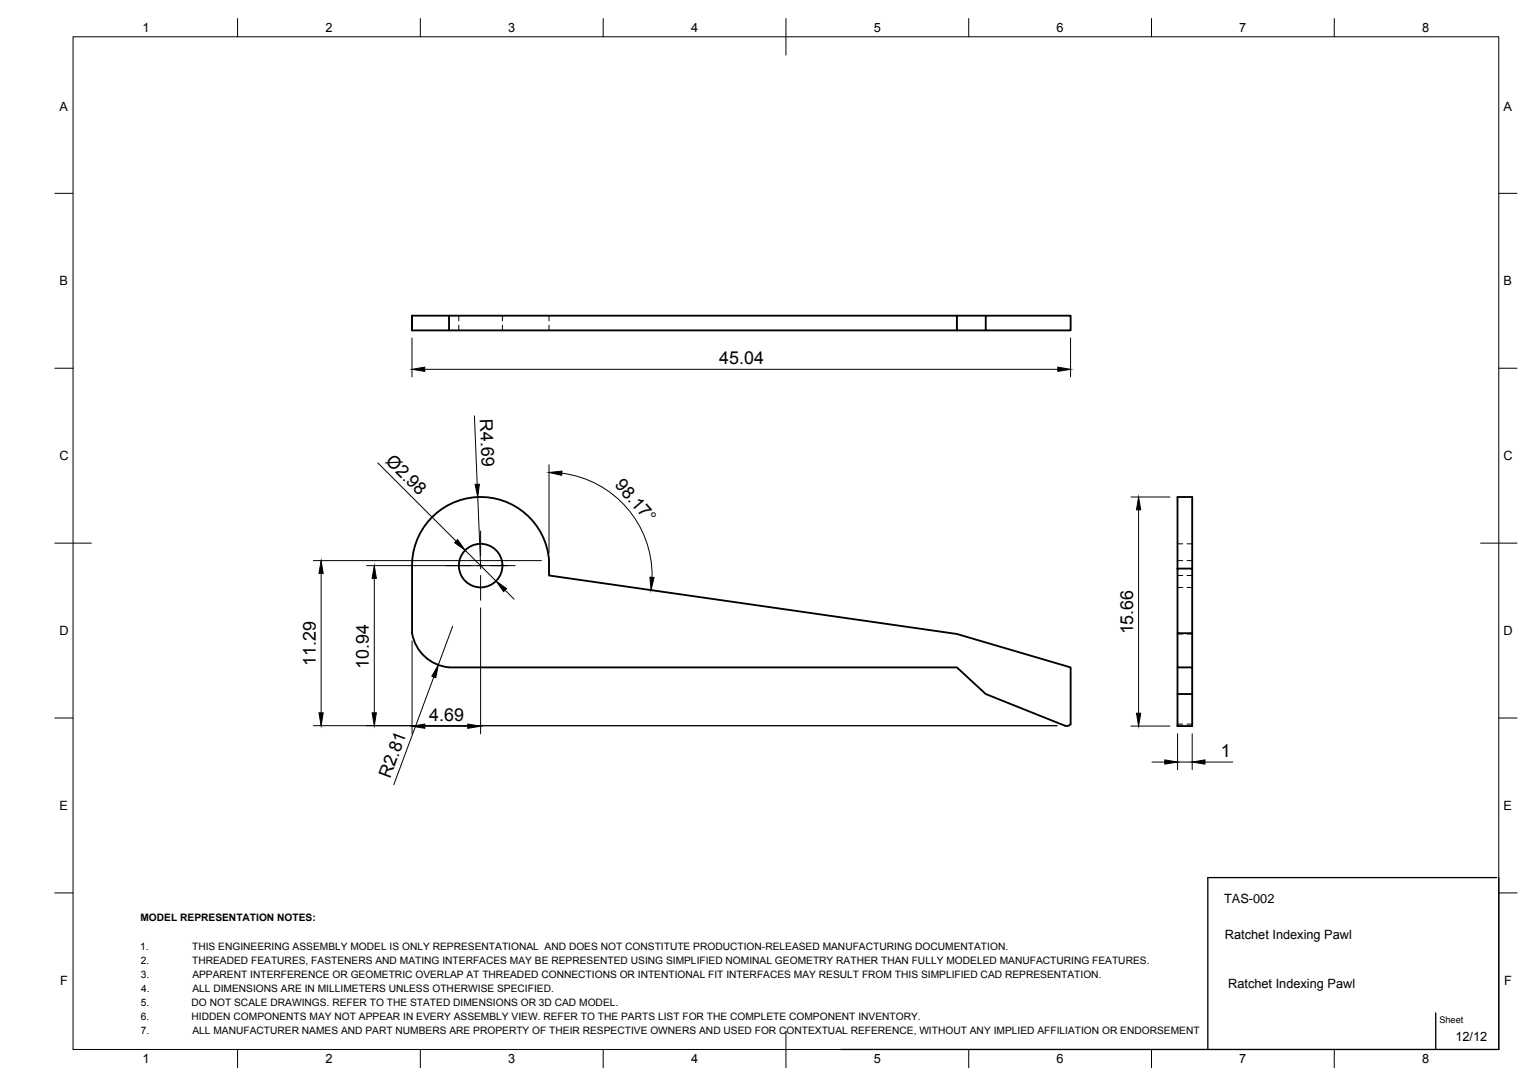
ISO-10303-21;
HEADER;
/* Generated by software containing ST-Developer
 * from STEP Tools, Inc. (www.steptools.com) 
 */

FILE_DESCRIPTION(
/* description */ ('STEP AP214'),
/* implementation_level */ '2;1');

FILE_NAME(
/* name */ 'Ratchet Indexing Pawl.step',
/* time_stamp */ '2026-11-04T19:38:14-08:00',
/* author */ (''),
/* organization */ (''),
/* preprocessor_version */ 'ST-DEVELOPER v20.2',
/* originating_system */ 'Autodesk Translation Framework v15.17.0.0',
/* authorisation */ '');

FILE_SCHEMA (('AUTOMOTIVE_DESIGN { 1 0 10303 214 3 1 1 }'));
ENDSEC;

DATA;
#10=MECHANICAL_DESIGN_GEOMETRIC_PRESENTATION_REPRESENTATION('',(#479),#36668);
#459=SHAPE_REPRESENTATION_RELATIONSHIP('SRR','None',#36715,#469);
#469=ADVANCED_BREP_SHAPE_REPRESENTATION('',(#488),#36667);
#479=STYLED_ITEM('',(#36766),#488);
#488=MANIFOLD_SOLID_BREP('Body1',#17803);
#772=CYLINDRICAL_SURFACE('',#19406,1.49172584788676);
#773=CYLINDRICAL_SURFACE('',#19410,4.6918515041613);
#774=CYLINDRICAL_SURFACE('',#19417,0.338583852498097);
#775=CYLINDRICAL_SURFACE('',#19423,2.81299719163292);
#971=FACE_BOUND('',#3583,.T.);
#972=FACE_BOUND('',#3585,.T.);
#1519=CIRCLE('',#19407,1.49172584788676);
#1520=CIRCLE('',#19408,1.49172584788676);
#1521=CIRCLE('',#19411,4.6918515041613);
#1522=CIRCLE('',#19412,4.6918515041613);
#1523=CIRCLE('',#19418,0.338583852498097);
#1524=CIRCLE('',#19419,0.338583852498097);
#1525=CIRCLE('',#19424,2.81299719163292);
#1526=CIRCLE('',#19425,2.81299719163292);
#2444=FACE_OUTER_BOUND('',#3570,.T.);
#2445=FACE_OUTER_BOUND('',#3571,.T.);
#2446=FACE_OUTER_BOUND('',#3572,.T.);
#2447=FACE_OUTER_BOUND('',#3573,.T.);
#2448=FACE_OUTER_BOUND('',#3574,.T.);
#2449=FACE_OUTER_BOUND('',#3575,.T.);
#2450=FACE_OUTER_BOUND('',#3576,.T.);
#2451=FACE_OUTER_BOUND('',#3577,.T.);
#2452=FACE_OUTER_BOUND('',#3578,.T.);
#2453=FACE_OUTER_BOUND('',#3579,.T.);
#2454=FACE_OUTER_BOUND('',#3580,.T.);
#2455=FACE_OUTER_BOUND('',#3581,.T.);
#2456=FACE_OUTER_BOUND('',#3582,.T.);
#2457=FACE_OUTER_BOUND('',#3584,.T.);
#3570=EDGE_LOOP('',(#16252,#16253,#16254,#16255));
#3571=EDGE_LOOP('',(#16256,#16257,#16258,#16259));
#3572=EDGE_LOOP('',(#16260,#16261,#16262,#16263));
#3573=EDGE_LOOP('',(#16264,#16265,#16266,#16267));
#3574=EDGE_LOOP('',(#16268,#16269,#16270,#16271));
#3575=EDGE_LOOP('',(#16272,#16273,#16274,#16275));
#3576=EDGE_LOOP('',(#16276,#16277,#16278,#16279));
#3577=EDGE_LOOP('',(#16280,#16281,#16282,#16283));
#3578=EDGE_LOOP('',(#16284,#16285,#16286,#16287));
#3579=EDGE_LOOP('',(#16288,#16289,#16290,#16291));
#3580=EDGE_LOOP('',(#16292,#16293,#16294,#16295));
#3581=EDGE_LOOP('',(#16296,#16297,#16298,#16299));
#3582=EDGE_LOOP('',(#16300,#16301,#16302,#16303,#16304,#16305,#16306,#16307,
#16308,#16309,#16310));
#3583=EDGE_LOOP('',(#16311));
#3584=EDGE_LOOP('',(#16312,#16313,#16314,#16315,#16316,#16317,#16318,#16319,
#16320,#16321,#16322));
#3585=EDGE_LOOP('',(#16323));
#5268=LINE('',#36565,#6978);
#5269=LINE('',#36570,#6979);
#5270=LINE('',#36572,#6980);
#5271=LINE('',#36574,#6981);
#5272=LINE('',#36575,#6982);
#5273=LINE('',#36580,#6983);
#5274=LINE('',#36584,#6984);
#5275=LINE('',#36586,#6985);
#5276=LINE('',#36587,#6986);
#5277=LINE('',#36590,#6987);
#5278=LINE('',#36592,#6988);
#5279=LINE('',#36593,#6989);
#5280=LINE('',#36596,#6990);
#5281=LINE('',#36598,#6991);
#5282=LINE('',#36599,#6992);
#5283=LINE('',#36602,#6993);
#5284=LINE('',#36604,#6994);
#5285=LINE('',#36605,#6995);
#5286=LINE('',#36611,#6996);
#5287=LINE('',#36614,#6997);
#5288=LINE('',#36616,#6998);
#5289=LINE('',#36617,#6999);
#5290=LINE('',#36620,#7000);
#5291=LINE('',#36622,#7001);
#5292=LINE('',#36623,#7002);
#5293=LINE('',#36626,#7003);
#5294=LINE('',#36628,#7004);
#5295=LINE('',#36629,#7005);
#6978=VECTOR('',#24106,1.49172584788676);
#6979=VECTOR('',#24111,1000.);
#6980=VECTOR('',#24112,1000.);
#6981=VECTOR('',#24113,1000.);
#6982=VECTOR('',#24114,1000.);
#6983=VECTOR('',#24119,1000.);
#6984=VECTOR('',#24124,1000.);
#6985=VECTOR('',#24125,1000.);
#6986=VECTOR('',#24126,1000.);
#6987=VECTOR('',#24129,1000.);
#6988=VECTOR('',#24130,1000.);
#6989=VECTOR('',#24131,1000.);
#6990=VECTOR('',#24134,1000.);
#6991=VECTOR('',#24135,1000.);
#6992=VECTOR('',#24136,1000.);
#6993=VECTOR('',#24139,1000.);
#6994=VECTOR('',#24140,1000.);
#6995=VECTOR('',#24141,1000.);
#6996=VECTOR('',#24148,1000.);
#6997=VECTOR('',#24151,1000.);
#6998=VECTOR('',#24152,1000.);
#6999=VECTOR('',#24153,1000.);
#7000=VECTOR('',#24156,1000.);
#7001=VECTOR('',#24157,1000.);
#7002=VECTOR('',#24158,1000.);
#7003=VECTOR('',#24161,1000.);
#7004=VECTOR('',#24162,1000.);
#7005=VECTOR('',#24163,1000.);
#8635=VERTEX_POINT('',#36562);
#8636=VERTEX_POINT('',#36564);
#8637=VERTEX_POINT('',#36568);
#8638=VERTEX_POINT('',#36569);
#8639=VERTEX_POINT('',#36571);
#8640=VERTEX_POINT('',#36573);
#8641=VERTEX_POINT('',#36577);
#8642=VERTEX_POINT('',#36579);
#8643=VERTEX_POINT('',#36583);
#8644=VERTEX_POINT('',#36585);
#8645=VERTEX_POINT('',#36589);
#8646=VERTEX_POINT('',#36591);
#8647=VERTEX_POINT('',#36595);
#8648=VERTEX_POINT('',#36597);
#8649=VERTEX_POINT('',#36601);
#8650=VERTEX_POINT('',#36603);
#8651=VERTEX_POINT('',#36607);
#8652=VERTEX_POINT('',#36609);
#8653=VERTEX_POINT('',#36613);
#8654=VERTEX_POINT('',#36615);
#8655=VERTEX_POINT('',#36619);
#8656=VERTEX_POINT('',#36621);
#8657=VERTEX_POINT('',#36625);
#8658=VERTEX_POINT('',#36627);
#11178=EDGE_CURVE('',#8635,#8635,#1519,.T.);
#11179=EDGE_CURVE('',#8635,#8636,#5268,.T.);
#11180=EDGE_CURVE('',#8636,#8636,#1520,.T.);
#11181=EDGE_CURVE('',#8637,#8638,#5269,.T.);
#11182=EDGE_CURVE('',#8639,#8638,#5270,.T.);
#11183=EDGE_CURVE('',#8640,#8639,#5271,.T.);
#11184=EDGE_CURVE('',#8640,#8637,#5272,.T.);
#11185=EDGE_CURVE('',#8641,#8640,#1521,.T.);
#11186=EDGE_CURVE('',#8641,#8642,#5273,.T.);
#11187=EDGE_CURVE('',#8642,#8637,#1522,.T.);
#11188=EDGE_CURVE('',#8643,#8642,#5274,.T.);
#11189=EDGE_CURVE('',#8644,#8641,#5275,.T.);
#11190=EDGE_CURVE('',#8644,#8643,#5276,.T.);
#11191=EDGE_CURVE('',#8645,#8643,#5277,.T.);
#11192=EDGE_CURVE('',#8646,#8644,#5278,.T.);
#11193=EDGE_CURVE('',#8646,#8645,#5279,.T.);
#11194=EDGE_CURVE('',#8647,#8645,#5280,.T.);
#11195=EDGE_CURVE('',#8648,#8646,#5281,.T.);
#11196=EDGE_CURVE('',#8648,#8647,#5282,.T.);
#11197=EDGE_CURVE('',#8649,#8647,#5283,.T.);
#11198=EDGE_CURVE('',#8650,#8648,#5284,.T.);
#11199=EDGE_CURVE('',#8650,#8649,#5285,.T.);
#11200=EDGE_CURVE('',#8651,#8649,#1523,.T.);
#11201=EDGE_CURVE('',#8652,#8650,#1524,.T.);
#11202=EDGE_CURVE('',#8652,#8651,#5286,.T.);
#11203=EDGE_CURVE('',#8653,#8651,#5287,.T.);
#11204=EDGE_CURVE('',#8654,#8652,#5288,.T.);
#11205=EDGE_CURVE('',#8654,#8653,#5289,.T.);
#11206=EDGE_CURVE('',#8655,#8653,#5290,.T.);
#11207=EDGE_CURVE('',#8656,#8654,#5291,.T.);
#11208=EDGE_CURVE('',#8656,#8655,#5292,.T.);
#11209=EDGE_CURVE('',#8657,#8655,#5293,.T.);
#11210=EDGE_CURVE('',#8658,#8656,#5294,.T.);
#11211=EDGE_CURVE('',#8658,#8657,#5295,.T.);
#11212=EDGE_CURVE('',#8638,#8657,#1525,.T.);
#11213=EDGE_CURVE('',#8639,#8658,#1526,.T.);
#16252=ORIENTED_EDGE('',*,*,#11178,.T.);
#16253=ORIENTED_EDGE('',*,*,#11179,.T.);
#16254=ORIENTED_EDGE('',*,*,#11180,.T.);
#16255=ORIENTED_EDGE('',*,*,#11179,.F.);
#16256=ORIENTED_EDGE('',*,*,#11181,.T.);
#16257=ORIENTED_EDGE('',*,*,#11182,.F.);
#16258=ORIENTED_EDGE('',*,*,#11183,.F.);
#16259=ORIENTED_EDGE('',*,*,#11184,.T.);
#16260=ORIENTED_EDGE('',*,*,#11185,.F.);
#16261=ORIENTED_EDGE('',*,*,#11186,.T.);
#16262=ORIENTED_EDGE('',*,*,#11187,.T.);
#16263=ORIENTED_EDGE('',*,*,#11184,.F.);
#16264=ORIENTED_EDGE('',*,*,#11188,.T.);
#16265=ORIENTED_EDGE('',*,*,#11186,.F.);
#16266=ORIENTED_EDGE('',*,*,#11189,.F.);
#16267=ORIENTED_EDGE('',*,*,#11190,.T.);
#16268=ORIENTED_EDGE('',*,*,#11191,.T.);
#16269=ORIENTED_EDGE('',*,*,#11190,.F.);
#16270=ORIENTED_EDGE('',*,*,#11192,.F.);
#16271=ORIENTED_EDGE('',*,*,#11193,.T.);
#16272=ORIENTED_EDGE('',*,*,#11194,.T.);
#16273=ORIENTED_EDGE('',*,*,#11193,.F.);
#16274=ORIENTED_EDGE('',*,*,#11195,.F.);
#16275=ORIENTED_EDGE('',*,*,#11196,.T.);
#16276=ORIENTED_EDGE('',*,*,#11197,.T.);
#16277=ORIENTED_EDGE('',*,*,#11196,.F.);
#16278=ORIENTED_EDGE('',*,*,#11198,.F.);
#16279=ORIENTED_EDGE('',*,*,#11199,.T.);
#16280=ORIENTED_EDGE('',*,*,#11200,.T.);
#16281=ORIENTED_EDGE('',*,*,#11199,.F.);
#16282=ORIENTED_EDGE('',*,*,#11201,.F.);
#16283=ORIENTED_EDGE('',*,*,#11202,.T.);
#16284=ORIENTED_EDGE('',*,*,#11203,.T.);
#16285=ORIENTED_EDGE('',*,*,#11202,.F.);
#16286=ORIENTED_EDGE('',*,*,#11204,.F.);
#16287=ORIENTED_EDGE('',*,*,#11205,.T.);
#16288=ORIENTED_EDGE('',*,*,#11206,.T.);
#16289=ORIENTED_EDGE('',*,*,#11205,.F.);
#16290=ORIENTED_EDGE('',*,*,#11207,.F.);
#16291=ORIENTED_EDGE('',*,*,#11208,.T.);
#16292=ORIENTED_EDGE('',*,*,#11209,.T.);
#16293=ORIENTED_EDGE('',*,*,#11208,.F.);
#16294=ORIENTED_EDGE('',*,*,#11210,.F.);
#16295=ORIENTED_EDGE('',*,*,#11211,.T.);
#16296=ORIENTED_EDGE('',*,*,#11212,.T.);
#16297=ORIENTED_EDGE('',*,*,#11211,.F.);
#16298=ORIENTED_EDGE('',*,*,#11213,.F.);
#16299=ORIENTED_EDGE('',*,*,#11182,.T.);
#16300=ORIENTED_EDGE('',*,*,#11212,.F.);
#16301=ORIENTED_EDGE('',*,*,#11181,.F.);
#16302=ORIENTED_EDGE('',*,*,#11187,.F.);
#16303=ORIENTED_EDGE('',*,*,#11188,.F.);
#16304=ORIENTED_EDGE('',*,*,#11191,.F.);
#16305=ORIENTED_EDGE('',*,*,#11194,.F.);
#16306=ORIENTED_EDGE('',*,*,#11197,.F.);
#16307=ORIENTED_EDGE('',*,*,#11200,.F.);
#16308=ORIENTED_EDGE('',*,*,#11203,.F.);
#16309=ORIENTED_EDGE('',*,*,#11206,.F.);
#16310=ORIENTED_EDGE('',*,*,#11209,.F.);
#16311=ORIENTED_EDGE('',*,*,#11178,.F.);
#16312=ORIENTED_EDGE('',*,*,#11213,.T.);
#16313=ORIENTED_EDGE('',*,*,#11210,.T.);
#16314=ORIENTED_EDGE('',*,*,#11207,.T.);
#16315=ORIENTED_EDGE('',*,*,#11204,.T.);
#16316=ORIENTED_EDGE('',*,*,#11201,.T.);
#16317=ORIENTED_EDGE('',*,*,#11198,.T.);
#16318=ORIENTED_EDGE('',*,*,#11195,.T.);
#16319=ORIENTED_EDGE('',*,*,#11192,.T.);
#16320=ORIENTED_EDGE('',*,*,#11189,.T.);
#16321=ORIENTED_EDGE('',*,*,#11185,.T.);
#16322=ORIENTED_EDGE('',*,*,#11183,.T.);
#16323=ORIENTED_EDGE('',*,*,#11180,.F.);
#16852=PLANE('',#19409);
#16853=PLANE('',#19413);
#16854=PLANE('',#19414);
#16855=PLANE('',#19415);
#16856=PLANE('',#19416);
#16857=PLANE('',#19420);
#16858=PLANE('',#19421);
#16859=PLANE('',#19422);
#16860=PLANE('',#19426);
#16861=PLANE('',#19427);
#17779=ADVANCED_FACE('',(#2444),#772,.F.);
#17780=ADVANCED_FACE('',(#2445),#16852,.F.);
#17781=ADVANCED_FACE('',(#2446),#773,.T.);
#17782=ADVANCED_FACE('',(#2447),#16853,.F.);
#17783=ADVANCED_FACE('',(#2448),#16854,.F.);
#17784=ADVANCED_FACE('',(#2449),#16855,.F.);
#17785=ADVANCED_FACE('',(#2450),#16856,.F.);
#17786=ADVANCED_FACE('',(#2451),#774,.T.);
#17787=ADVANCED_FACE('',(#2452),#16857,.F.);
#17788=ADVANCED_FACE('',(#2453),#16858,.F.);
#17789=ADVANCED_FACE('',(#2454),#16859,.F.);
#17790=ADVANCED_FACE('',(#2455),#775,.T.);
#17791=ADVANCED_FACE('',(#2456,#971),#16860,.T.);
#17792=ADVANCED_FACE('',(#2457,#972),#16861,.F.);
#17803=CLOSED_SHELL('',(#17779,#17780,#17781,#17782,#17783,#17784,#17785,
#17786,#17787,#17788,#17789,#17790,#17791,#17792));
#19405=AXIS2_PLACEMENT_3D('',#36560,#24100,#24101);
#19406=AXIS2_PLACEMENT_3D('',#36561,#24102,#24103);
#19407=AXIS2_PLACEMENT_3D('',#36563,#24104,#24105);
#19408=AXIS2_PLACEMENT_3D('',#36566,#24107,#24108);
#19409=AXIS2_PLACEMENT_3D('',#36567,#24109,#24110);
#19410=AXIS2_PLACEMENT_3D('',#36576,#24115,#24116);
#19411=AXIS2_PLACEMENT_3D('',#36578,#24117,#24118);
#19412=AXIS2_PLACEMENT_3D('',#36581,#24120,#24121);
#19413=AXIS2_PLACEMENT_3D('',#36582,#24122,#24123);
#19414=AXIS2_PLACEMENT_3D('',#36588,#24127,#24128);
#19415=AXIS2_PLACEMENT_3D('',#36594,#24132,#24133);
#19416=AXIS2_PLACEMENT_3D('',#36600,#24137,#24138);
#19417=AXIS2_PLACEMENT_3D('',#36606,#24142,#24143);
#19418=AXIS2_PLACEMENT_3D('',#36608,#24144,#24145);
#19419=AXIS2_PLACEMENT_3D('',#36610,#24146,#24147);
#19420=AXIS2_PLACEMENT_3D('',#36612,#24149,#24150);
#19421=AXIS2_PLACEMENT_3D('',#36618,#24154,#24155);
#19422=AXIS2_PLACEMENT_3D('',#36624,#24159,#24160);
#19423=AXIS2_PLACEMENT_3D('',#36630,#24164,#24165);
#19424=AXIS2_PLACEMENT_3D('',#36631,#24166,#24167);
#19425=AXIS2_PLACEMENT_3D('',#36632,#24168,#24169);
#19426=AXIS2_PLACEMENT_3D('',#36633,#24170,#24171);
#19427=AXIS2_PLACEMENT_3D('',#36634,#24172,#24173);
#24100=DIRECTION('axis',(0.,0.,1.));
#24101=DIRECTION('refdir',(1.,0.,0.));
#24102=DIRECTION('center_axis',(0.,0.,-1.));
#24103=DIRECTION('ref_axis',(-1.,0.,0.));
#24104=DIRECTION('center_axis',(0.,0.,1.));
#24105=DIRECTION('ref_axis',(1.,0.,0.));
#24106=DIRECTION('',(0.,0.,-1.));
#24107=DIRECTION('center_axis',(0.,0.,-1.));
#24108=DIRECTION('ref_axis',(-1.,0.,0.));
#24109=DIRECTION('center_axis',(-0.999428214444506,-0.033811893946752,0.));
#24110=DIRECTION('ref_axis',(-0.033811893946752,0.999428214444506,0.));
#24111=DIRECTION('',(0.033811893946752,-0.999428214444506,0.));
#24112=DIRECTION('',(0.,0.,1.));
#24113=DIRECTION('',(0.033811893946752,-0.999428214444506,0.));
#24114=DIRECTION('',(0.,0.,1.));
#24115=DIRECTION('center_axis',(0.,0.,1.));
#24116=DIRECTION('ref_axis',(0.999428214444506,0.0338118939467526,0.));
#24117=DIRECTION('center_axis',(0.,0.,-1.));
#24118=DIRECTION('ref_axis',(0.999428214444506,0.0338118939467526,0.));
#24119=DIRECTION('',(0.,0.,1.));
#24120=DIRECTION('center_axis',(0.,0.,-1.));
#24121=DIRECTION('ref_axis',(0.999428214444506,0.0338118939467526,0.));
#24122=DIRECTION('center_axis',(0.999428214444506,0.0338118939467537,0.));
#24123=DIRECTION('ref_axis',(0.,0.,-1.));
#24124=DIRECTION('',(-0.0338118939467537,0.999428214444506,0.));
#24125=DIRECTION('',(-0.0338118939467537,0.999428214444506,0.));
#24126=DIRECTION('',(0.,0.,1.));
#24127=DIRECTION('center_axis',(0.175442327597817,-0.984489710300245,0.));
#24128=DIRECTION('ref_axis',(0.984489710300245,0.175442327597816,0.));
#24129=DIRECTION('',(0.984489710300245,0.175442327597816,0.));
#24130=DIRECTION('',(0.984489710300248,0.1754423275978,0.));
#24131=DIRECTION('',(0.,0.,1.));
#24132=DIRECTION('center_axis',(0.314024880544539,-0.949414753624036,0.));
#24133=DIRECTION('ref_axis',(0.949414753624036,0.314024880544539,0.));
#24134=DIRECTION('',(0.949414753624036,0.314024880544539,0.));
#24135=DIRECTION('',(0.949414753624036,0.314024880544539,0.));
#24136=DIRECTION('',(0.,0.,1.));
#24137=DIRECTION('center_axis',(0.999428214444506,0.033811893946752,0.));
#24138=DIRECTION('ref_axis',(0.,0.,-1.));
#24139=DIRECTION('',(-0.033811893946752,0.999428214444506,0.));
#24140=DIRECTION('',(-0.033811893946752,0.999428214444506,0.));
#24141=DIRECTION('',(0.,0.,1.));
#24142=DIRECTION('center_axis',(0.,0.,1.));
#24143=DIRECTION('ref_axis',(0.999428214444506,0.0338118939467424,0.));
#24144=DIRECTION('center_axis',(0.,0.,-1.));
#24145=DIRECTION('ref_axis',(0.999428214444506,0.0338118939467424,0.));
#24146=DIRECTION('center_axis',(0.,0.,-1.));
#24147=DIRECTION('ref_axis',(0.999428214444506,0.0338118939467424,0.));
#24148=DIRECTION('',(0.,0.,1.));
#24149=DIRECTION('center_axis',(-0.40290063302029,0.915243727054084,0.));
#24150=DIRECTION('ref_axis',(0.,0.,1.));
#24151=DIRECTION('',(-0.915243727054084,-0.402900633020289,0.));
#24152=DIRECTION('',(-0.915243727054084,-0.402900633020289,0.));
#24153=DIRECTION('',(0.,0.,1.));
#24154=DIRECTION('center_axis',(-0.702321846847344,0.711859553171084,0.));
#24155=DIRECTION('ref_axis',(0.,0.,1.));
#24156=DIRECTION('',(-0.711859553171084,-0.702321846847344,0.));
#24157=DIRECTION('',(-0.711859553171084,-0.702321846847344,0.));
#24158=DIRECTION('',(0.,0.,1.));
#24159=DIRECTION('center_axis',(-0.033811893946752,0.999428214444506,0.));
#24160=DIRECTION('ref_axis',(-0.999428214444506,-0.033811893946752,0.));
#24161=DIRECTION('',(-0.999428214444506,-0.033811893946752,0.));
#24162=DIRECTION('',(-0.999428214444506,-0.033811893946752,0.));
#24163=DIRECTION('',(0.,0.,1.));
#24164=DIRECTION('center_axis',(0.,0.,1.));
#24165=DIRECTION('ref_axis',(0.999428214444506,0.0338118939467518,0.));
#24166=DIRECTION('center_axis',(0.,0.,-1.));
#24167=DIRECTION('ref_axis',(0.999428214444506,0.0338118939467518,0.));
#24168=DIRECTION('center_axis',(0.,0.,-1.));
#24169=DIRECTION('ref_axis',(0.999428214444506,0.0338118939467518,0.));
#24170=DIRECTION('center_axis',(0.,0.,1.));
#24171=DIRECTION('ref_axis',(0.033811893946752,-0.999428214444506,0.));
#24172=DIRECTION('center_axis',(0.,0.,1.));
#24173=DIRECTION('ref_axis',(0.033811893946752,-0.999428214444506,0.));
#36560=CARTESIAN_POINT('',(0.,0.,0.));
#36561=CARTESIAN_POINT('Origin',(19.9513700273636,43.5818784659284,216.094898865397));
#36562=CARTESIAN_POINT('',(21.4430958752503,43.5818784659284,209.094898865397));
#36563=CARTESIAN_POINT('Origin',(19.9513700273636,43.5818784659284,209.094898865397));
#36564=CARTESIAN_POINT('',(21.4430958752503,43.5818784659284,208.094898865397));
#36565=CARTESIAN_POINT('',(21.4430958752503,43.5818784659284,216.094898865397));
#36566=CARTESIAN_POINT('Origin',(19.9513700273636,43.5818784659284,208.094898865397));
#36567=CARTESIAN_POINT('Origin',(24.6430224985391,43.5386624163653,208.094898865397));
#36568=CARTESIAN_POINT('',(24.6430224985391,43.5386624163653,209.094898865397));
#36569=CARTESIAN_POINT('',(24.7923296637165,39.1253694570289,209.094898865397));
#36570=CARTESIAN_POINT('',(24.6430224985391,43.5386624163653,209.094898865397));
#36571=CARTESIAN_POINT('',(24.7923296637165,39.1253694570289,208.094898865397));
#36572=CARTESIAN_POINT('',(24.7923296637165,39.1253694570289,208.094898865397));
#36573=CARTESIAN_POINT('',(24.6430224985391,43.5386624163653,208.094898865397));
#36574=CARTESIAN_POINT('',(24.6430224985391,43.5386624163653,208.094898865397));
#36575=CARTESIAN_POINT('',(24.6430224985391,43.5386624163653,208.094898865397));
#36576=CARTESIAN_POINT('Origin',(19.951370027377,43.5818784659222,208.094898865397));
#36577=CARTESIAN_POINT('',(15.2632338299238,43.7685587574091,208.094898865397));
#36578=CARTESIAN_POINT('Origin',(19.951370027377,43.5818784659222,208.094898865397));
#36579=CARTESIAN_POINT('',(15.2632338299238,43.7685587574091,209.094898865397));
#36580=CARTESIAN_POINT('',(15.2632338299238,43.7685587574091,208.094898865397));
#36581=CARTESIAN_POINT('Origin',(19.951370027377,43.5818784659222,209.094898865397));
#36582=CARTESIAN_POINT('Origin',(15.2976067234458,42.7525482478522,208.094898865397));
#36583=CARTESIAN_POINT('',(15.2976067234458,42.7525482478522,209.094898865397));
#36584=CARTESIAN_POINT('',(15.2976067234458,42.7525482478522,209.094898865397));
#36585=CARTESIAN_POINT('',(15.2976067234458,42.7525482478522,208.094898865397));
#36586=CARTESIAN_POINT('',(15.2976067234458,42.7525482478522,208.094898865397));
#36587=CARTESIAN_POINT('',(15.2976067234458,42.7525482478522,208.094898865397));
#36588=CARTESIAN_POINT('Origin',(-2.17548604454373,39.6387319900736,208.094898865397));
#36589=CARTESIAN_POINT('',(-12.4435067339657,37.8089053999865,209.094898865397));
#36590=CARTESIAN_POINT('',(-2.17548604454373,39.6387319900736,209.094898865397));
#36591=CARTESIAN_POINT('',(-12.4435067339657,37.8089053999865,208.094898865397));
#36592=CARTESIAN_POINT('',(-12.4435067339657,37.8089053999865,208.094898865397));
#36593=CARTESIAN_POINT('',(-12.4435067339657,37.8089053999865,208.094898865397));
#36594=CARTESIAN_POINT('Origin',(-20.1379345336707,35.2639251777624,208.094898865397));
#36595=CARTESIAN_POINT('',(-20.1379345336707,35.2639251777624,209.094898865397));
#36596=CARTESIAN_POINT('',(-20.1379345336707,35.2639251777624,209.094898865397));
#36597=CARTESIAN_POINT('',(-20.1379345336707,35.2639251777624,208.094898865397));
#36598=CARTESIAN_POINT('',(-20.1379345336707,35.2639251777624,208.094898865397));
#36599=CARTESIAN_POINT('',(-20.1379345336707,35.2639251777624,208.094898865397));
#36600=CARTESIAN_POINT('Origin',(-20.0067099032547,31.3851244730677,208.094898865397));
#36601=CARTESIAN_POINT('',(-20.0067099032547,31.3851244730677,209.094898865397));
#36602=CARTESIAN_POINT('',(-20.0067099032547,31.3851244730677,209.094898865397));
#36603=CARTESIAN_POINT('',(-20.0067099032547,31.3851244730677,208.094898865397));
#36604=CARTESIAN_POINT('',(-20.0067099032547,31.3851244730677,208.094898865397));
#36605=CARTESIAN_POINT('',(-20.0067099032547,31.3851244730677,208.094898865397));
#36606=CARTESIAN_POINT('Origin',(-19.7470473101411,31.6024131357033,208.094898865397));
#36607=CARTESIAN_POINT('',(-19.6054127952646,31.2948766510902,209.094898865397));
#36608=CARTESIAN_POINT('Origin',(-19.7470473101411,31.6024131357033,209.094898865397));
#36609=CARTESIAN_POINT('',(-19.6054127952646,31.2948766510902,208.094898865397));
#36610=CARTESIAN_POINT('Origin',(-19.7470473101411,31.6024131357033,208.094898865397));
#36611=CARTESIAN_POINT('',(-19.6054127952646,31.2948766510902,208.094898865397));
#36612=CARTESIAN_POINT('Origin',(-14.2756540048791,33.64109670922,208.094898865397));
#36613=CARTESIAN_POINT('',(-14.2756540048791,33.64109670922,209.094898865397));
#36614=CARTESIAN_POINT('',(-14.2756540048791,33.64109670922,209.094898865397));
#36615=CARTESIAN_POINT('',(-14.2756540048791,33.64109670922,208.094898865397));
#36616=CARTESIAN_POINT('',(-14.2756540048791,33.64109670922,208.094898865397));
#36617=CARTESIAN_POINT('',(-14.2756540048791,33.64109670922,208.094898865397));
#36618=CARTESIAN_POINT('Origin',(-12.364689956501,35.5264570920893,208.094898865397));
#36619=CARTESIAN_POINT('',(-12.364689956501,35.5264570920893,209.094898865397));
#36620=CARTESIAN_POINT('',(-12.364689956501,35.5264570920893,209.094898865397));
#36621=CARTESIAN_POINT('',(-12.364689956501,35.5264570920893,208.094898865397));
#36622=CARTESIAN_POINT('',(-12.364689956501,35.5264570920893,208.094898865397));
#36623=CARTESIAN_POINT('',(-12.364689956501,35.5264570920893,208.094898865397));
#36624=CARTESIAN_POINT('Origin',(22.3452540862996,36.7007374755235,208.094898865397));
#36625=CARTESIAN_POINT('',(22.3452540862996,36.7007374755235,209.094898865397));
#36626=CARTESIAN_POINT('',(22.3452540862996,36.7007374755235,209.094898865397));
#36627=CARTESIAN_POINT('',(22.3452540862996,36.7007374755235,208.094898865397));
#36628=CARTESIAN_POINT('',(22.3452540862996,36.7007374755235,208.094898865397));
#36629=CARTESIAN_POINT('',(22.3452540862996,36.7007374755235,208.094898865397));
#36630=CARTESIAN_POINT('Origin',(22.0034443343711,39.4928906399508,208.094898865397));
#36631=CARTESIAN_POINT('Origin',(22.0034443343711,39.4928906399508,209.094898865397));
#36632=CARTESIAN_POINT('Origin',(22.0034443343711,39.4928906399508,208.094898865397));
#36633=CARTESIAN_POINT('Origin',(22.0034443343711,39.4928906399508,209.094898865397));
#36634=CARTESIAN_POINT('Origin',(22.0034443343711,39.4928906399508,208.094898865397));
#36655=UNCERTAINTY_MEASURE_WITH_UNIT(LENGTH_MEASURE(0.01),#36669,
'DISTANCE_ACCURACY_VALUE',
'Maximum model space distance between geometric entities at asserted c
onnectivities');
#36656=UNCERTAINTY_MEASURE_WITH_UNIT(LENGTH_MEASURE(0.01),#36669,
'DISTANCE_ACCURACY_VALUE',
'Maximum model space distance between geometric entities at asserted c
onnectivities');
#36667=(
GEOMETRIC_REPRESENTATION_CONTEXT(3)
GLOBAL_UNCERTAINTY_ASSIGNED_CONTEXT((#36655))
GLOBAL_UNIT_ASSIGNED_CONTEXT((#36669,#36671,#36672))
REPRESENTATION_CONTEXT('','3D')
);
#36668=(
GEOMETRIC_REPRESENTATION_CONTEXT(3)
GLOBAL_UNCERTAINTY_ASSIGNED_CONTEXT((#36656))
GLOBAL_UNIT_ASSIGNED_CONTEXT((#36669,#36671,#36672))
REPRESENTATION_CONTEXT('','3D')
);
#36669=(
LENGTH_UNIT()
NAMED_UNIT(*)
SI_UNIT(.MILLI.,.METRE.)
);
#36671=(
NAMED_UNIT(*)
PLANE_ANGLE_UNIT()
SI_UNIT($,.RADIAN.)
);
#36672=(
NAMED_UNIT(*)
SI_UNIT($,.STERADIAN.)
SOLID_ANGLE_UNIT()
);
#36683=SHAPE_DEFINITION_REPRESENTATION(#36694,#36715);
#36694=PRODUCT_DEFINITION_SHAPE('',$,#36727);
#36715=SHAPE_REPRESENTATION('',(#19405),#36667);
#36716=PRODUCT_DEFINITION_CONTEXT('part definition',#36751,'design');
#36727=PRODUCT_DEFINITION('Ratchet Indexing Pawl',
'Ratchet Indexing Pawl',#36738,#36716);
#36738=PRODUCT_DEFINITION_FORMATION('',$,#36763);
#36751=APPLICATION_CONTEXT(
'Core Data for Automotive Mechanical Design Process');
#36752=PRODUCT_CONTEXT('part definition',#36751,'mechanical');
#36763=PRODUCT('Ratchet Indexing Pawl','Ratchet Indexing Pawl',$,(#36752));
#36766=PRESENTATION_STYLE_ASSIGNMENT((#36773));
#36773=SURFACE_STYLE_USAGE(.BOTH.,#36780);
#36780=SURFACE_SIDE_STYLE('',(#36787));
#36787=SURFACE_STYLE_FILL_AREA(#36794);
#36794=FILL_AREA_STYLE('Opaque(104,114,127)',(#36801));
#36801=FILL_AREA_STYLE_COLOUR('Opaque(104,114,127)',#36808);
#36808=COLOUR_RGB('Opaque(104,114,127)',0.407843137254902,0.447058823529412,
0.498039215686275);
ENDSEC;
END-ISO-10303-21;
